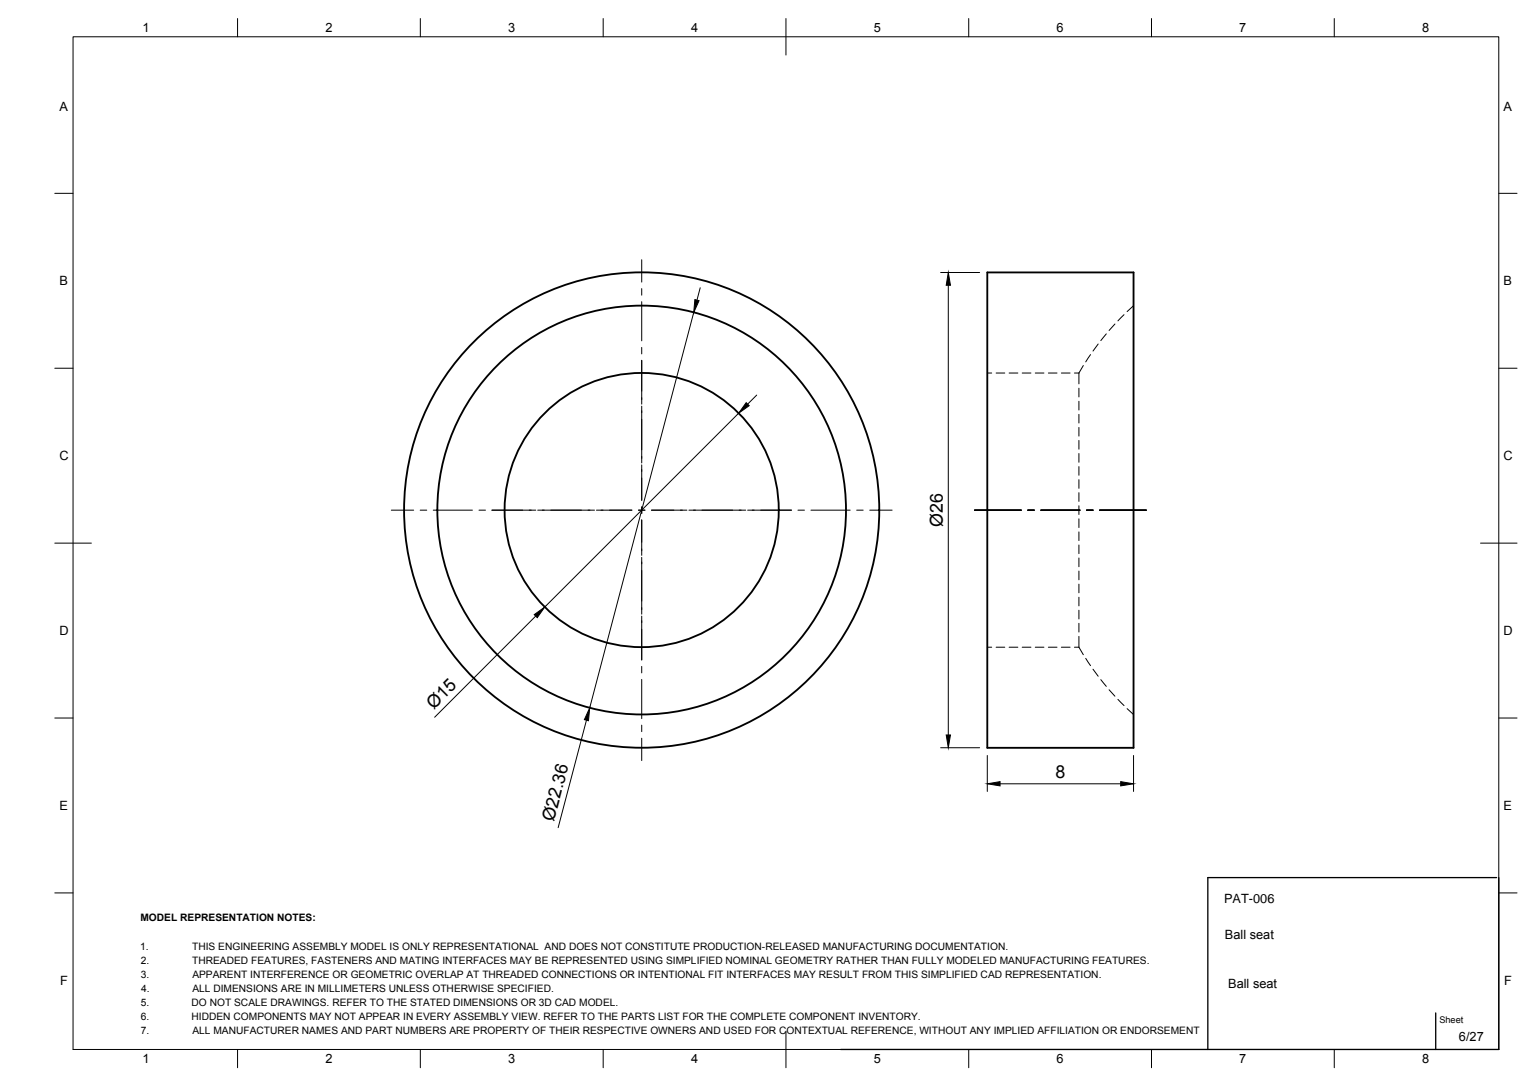
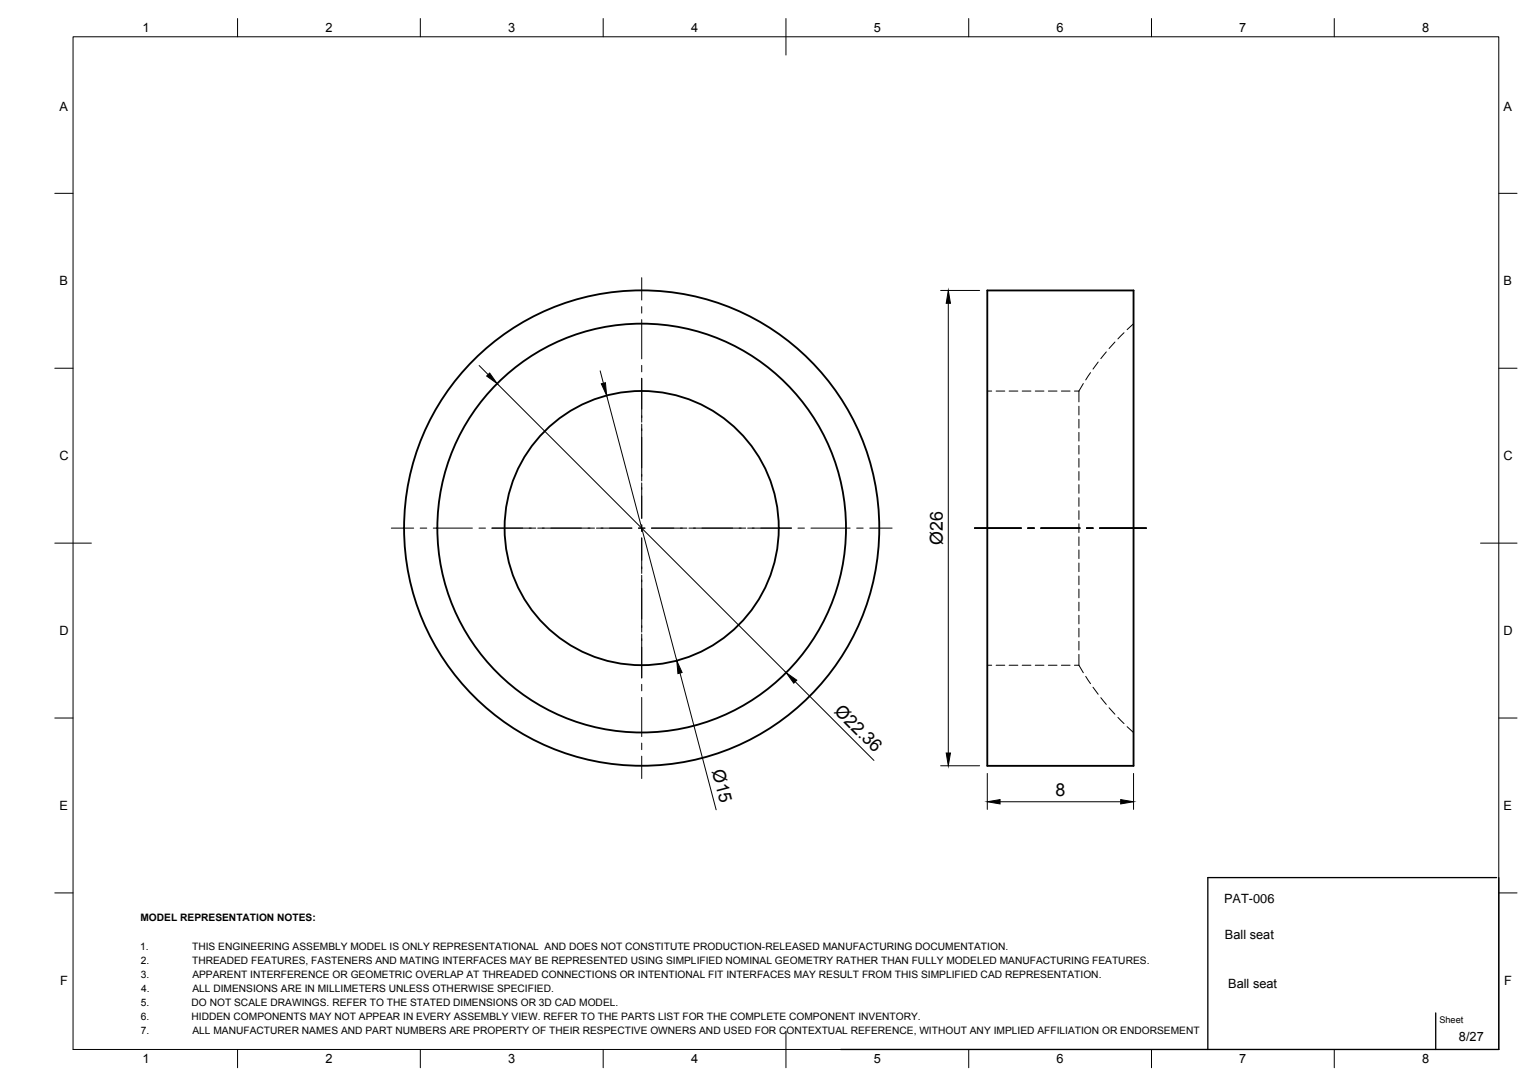
ISO-10303-21;
HEADER;
/* Generated by software containing ST-Developer
 * from STEP Tools, Inc. (www.steptools.com) 
 */

FILE_DESCRIPTION(
/* description */ ('Ball-type isolation valve (generic)'),
/* implementation_level */ '2;1');

FILE_NAME(
/* name */ 'Ball seat.step',
/* time_stamp */ '2026-10-27T10:53:05-07:00',
/* author */ (''),
/* organization */ (''),
/* preprocessor_version */ 'ST-DEVELOPER v20.2',
/* originating_system */ 'Autodesk Translation Framework v15.17.0.0',
/* authorisation */ '');

FILE_SCHEMA (('AUTOMOTIVE_DESIGN { 1 0 10303 214 3 1 1 }'));
ENDSEC;

DATA;
#10=MECHANICAL_DESIGN_GEOMETRIC_PRESENTATION_REPRESENTATION('',(#278),#7425);
#226=SHAPE_REPRESENTATION_RELATIONSHIP('SRR','None',#7536,#252);
#252=ADVANCED_BREP_SHAPE_REPRESENTATION('',(#304),#7399);
#278=STYLED_ITEM('',(#7730),#304);
#304=MANIFOLD_SOLID_BREP('Body1',#4083);
#327=SPHERICAL_SURFACE('',#4444,1.5);
#345=FACE_BOUND('',#864,.T.);
#346=FACE_BOUND('',#868,.T.);
#347=FACE_BOUND('',#870,.T.);
#430=PLANE('',#4452);
#431=PLANE('',#4453);
#600=FACE_OUTER_BOUND('',#863,.T.);
#601=FACE_OUTER_BOUND('',#865,.T.);
#602=FACE_OUTER_BOUND('',#866,.T.);
#603=FACE_OUTER_BOUND('',#867,.T.);
#604=FACE_OUTER_BOUND('',#869,.T.);
#863=EDGE_LOOP('',(#2867));
#864=EDGE_LOOP('',(#2868));
#865=EDGE_LOOP('',(#2869,#2870,#2871,#2872));
#866=EDGE_LOOP('',(#2873,#2874,#2875,#2876));
#867=EDGE_LOOP('',(#2877));
#868=EDGE_LOOP('',(#2878));
#869=EDGE_LOOP('',(#2879));
#870=EDGE_LOOP('',(#2880));
#1190=LINE('',#6309,#1498);
#1191=LINE('',#6315,#1499);
#1498=VECTOR('',#5021,0.75);
#1499=VECTOR('',#5028,1.3);
#1802=CIRCLE('',#4445,1.11803398874989);
#1803=CIRCLE('',#4446,0.75);
#1804=CIRCLE('',#4448,0.75);
#1805=CIRCLE('',#4450,1.3);
#1806=CIRCLE('',#4451,1.3);
#1987=VERTEX_POINT('',#6303);
#1988=VERTEX_POINT('',#6305);
#1989=VERTEX_POINT('',#6308);
#1990=VERTEX_POINT('',#6312);
#1991=VERTEX_POINT('',#6314);
#2326=EDGE_CURVE('',#1987,#1987,#1802,.T.);
#2327=EDGE_CURVE('',#1988,#1988,#1803,.T.);
#2328=EDGE_CURVE('',#1988,#1989,#1190,.T.);
#2329=EDGE_CURVE('',#1989,#1989,#1804,.T.);
#2330=EDGE_CURVE('',#1990,#1990,#1805,.T.);
#2331=EDGE_CURVE('',#1990,#1991,#1191,.T.);
#2332=EDGE_CURVE('',#1991,#1991,#1806,.T.);
#2867=ORIENTED_EDGE('',*,*,#2326,.F.);
#2868=ORIENTED_EDGE('',*,*,#2327,.F.);
#2869=ORIENTED_EDGE('',*,*,#2327,.T.);
#2870=ORIENTED_EDGE('',*,*,#2328,.T.);
#2871=ORIENTED_EDGE('',*,*,#2329,.T.);
#2872=ORIENTED_EDGE('',*,*,#2328,.F.);
#2873=ORIENTED_EDGE('',*,*,#2330,.F.);
#2874=ORIENTED_EDGE('',*,*,#2331,.T.);
#2875=ORIENTED_EDGE('',*,*,#2332,.T.);
#2876=ORIENTED_EDGE('',*,*,#2331,.F.);
#2877=ORIENTED_EDGE('',*,*,#2330,.T.);
#2878=ORIENTED_EDGE('',*,*,#2326,.T.);
#2879=ORIENTED_EDGE('',*,*,#2332,.F.);
#2880=ORIENTED_EDGE('',*,*,#2329,.F.);
#3774=CYLINDRICAL_SURFACE('',#4447,0.75);
#3775=CYLINDRICAL_SURFACE('',#4449,1.3);
#3854=ADVANCED_FACE('',(#600,#345),#327,.F.);
#3855=ADVANCED_FACE('',(#601),#3774,.F.);
#3856=ADVANCED_FACE('',(#602),#3775,.T.);
#3857=ADVANCED_FACE('',(#603,#346),#430,.T.);
#3858=ADVANCED_FACE('',(#604,#347),#431,.F.);
#4083=CLOSED_SHELL('',(#3854,#3855,#3856,#3857,#3858));
#4443=AXIS2_PLACEMENT_3D('',#6301,#5011,#5012);
#4444=AXIS2_PLACEMENT_3D('',#6302,#5013,#5014);
#4445=AXIS2_PLACEMENT_3D('',#6304,#5015,#5016);
#4446=AXIS2_PLACEMENT_3D('',#6306,#5017,#5018);
#4447=AXIS2_PLACEMENT_3D('',#6307,#5019,#5020);
#4448=AXIS2_PLACEMENT_3D('',#6310,#5022,#5023);
#4449=AXIS2_PLACEMENT_3D('',#6311,#5024,#5025);
#4450=AXIS2_PLACEMENT_3D('',#6313,#5026,#5027);
#4451=AXIS2_PLACEMENT_3D('',#6316,#5029,#5030);
#4452=AXIS2_PLACEMENT_3D('',#6317,#5031,#5032);
#4453=AXIS2_PLACEMENT_3D('',#6318,#5033,#5034);
#5011=DIRECTION('axis',(0.,0.,1.));
#5012=DIRECTION('refdir',(1.,0.,0.));
#5013=DIRECTION('center_axis',(6.12323399573677E-17,0.,1.));
#5014=DIRECTION('ref_axis',(1.,0.,0.));
#5015=DIRECTION('center_axis',(0.,-1.,0.));
#5016=DIRECTION('ref_axis',(0.,0.,-1.));
#5017=DIRECTION('center_axis',(0.,1.,0.));
#5018=DIRECTION('ref_axis',(1.,0.,0.));
#5019=DIRECTION('center_axis',(0.,1.,0.));
#5020=DIRECTION('ref_axis',(1.,0.,0.));
#5021=DIRECTION('',(0.,-1.,0.));
#5022=DIRECTION('center_axis',(0.,-1.,0.));
#5023=DIRECTION('ref_axis',(1.,0.,0.));
#5024=DIRECTION('center_axis',(0.,1.,0.));
#5025=DIRECTION('ref_axis',(1.,0.,0.));
#5026=DIRECTION('center_axis',(0.,1.,0.));
#5027=DIRECTION('ref_axis',(1.,0.,0.));
#5028=DIRECTION('',(0.,-1.,0.));
#5029=DIRECTION('center_axis',(0.,1.,0.));
#5030=DIRECTION('ref_axis',(1.,0.,0.));
#5031=DIRECTION('center_axis',(0.,1.,0.));
#5032=DIRECTION('ref_axis',(1.,0.,0.));
#5033=DIRECTION('center_axis',(0.,1.,0.));
#5034=DIRECTION('ref_axis',(1.,0.,0.));
#6301=CARTESIAN_POINT('',(0.,0.,0.));
#6302=CARTESIAN_POINT('Origin',(0.,0.,5.));
#6303=CARTESIAN_POINT('',(-1.36919674566051E-16,-1.,6.11803398874989));
#6304=CARTESIAN_POINT('Origin',(0.,-1.,5.));
#6305=CARTESIAN_POINT('',(-0.75,-1.29903810567666,5.));
#6306=CARTESIAN_POINT('Origin',(0.,-1.29903810567666,5.));
#6307=CARTESIAN_POINT('Origin',(0.,-1.8,5.));
#6308=CARTESIAN_POINT('',(-0.75,-1.8,5.));
#6309=CARTESIAN_POINT('',(-0.75,-1.8,5.));
#6310=CARTESIAN_POINT('Origin',(0.,-1.8,5.));
#6311=CARTESIAN_POINT('Origin',(0.,-1.8,5.));
#6312=CARTESIAN_POINT('',(-1.3,-1.,5.));
#6313=CARTESIAN_POINT('Origin',(0.,-1.,5.));
#6314=CARTESIAN_POINT('',(-1.3,-1.8,5.));
#6315=CARTESIAN_POINT('',(-1.3,-1.8,5.));
#6316=CARTESIAN_POINT('Origin',(0.,-1.8,5.));
#6317=CARTESIAN_POINT('Origin',(0.,-1.,5.));
#6318=CARTESIAN_POINT('Origin',(0.,-1.8,5.));
#7369=UNCERTAINTY_MEASURE_WITH_UNIT(LENGTH_MEASURE(0.001),#7426,
'DISTANCE_ACCURACY_VALUE',
'Maximum model space distance between geometric entities at asserted c
onnectivities');
#7395=UNCERTAINTY_MEASURE_WITH_UNIT(LENGTH_MEASURE(0.001),#7426,
'DISTANCE_ACCURACY_VALUE',
'Maximum model space distance between geometric entities at asserted c
onnectivities');
#7399=(
GEOMETRIC_REPRESENTATION_CONTEXT(3)
GLOBAL_UNCERTAINTY_ASSIGNED_CONTEXT((#7369))
GLOBAL_UNIT_ASSIGNED_CONTEXT((#7426,#7428,#7429))
REPRESENTATION_CONTEXT('','3D')
);
#7425=(
GEOMETRIC_REPRESENTATION_CONTEXT(3)
GLOBAL_UNCERTAINTY_ASSIGNED_CONTEXT((#7395))
GLOBAL_UNIT_ASSIGNED_CONTEXT((#7426,#7428,#7429))
REPRESENTATION_CONTEXT('','3D')
);
#7426=(
LENGTH_UNIT()
NAMED_UNIT(*)
SI_UNIT(.CENTI.,.METRE.)
);
#7428=(
NAMED_UNIT(*)
PLANE_ANGLE_UNIT()
SI_UNIT($,.RADIAN.)
);
#7429=(
NAMED_UNIT(*)
SI_UNIT($,.STERADIAN.)
SOLID_ANGLE_UNIT()
);
#7433=SHAPE_DEFINITION_REPRESENTATION(#7462,#7536);
#7462=PRODUCT_DEFINITION_SHAPE('',$,#7566);
#7536=SHAPE_REPRESENTATION('',(#4443),#7399);
#7562=PRODUCT_DEFINITION_CONTEXT('part definition',#7651,'design');
#7566=PRODUCT_DEFINITION('Ball seat','Ball seat',#7595,#7562);
#7595=PRODUCT_DEFINITION_FORMATION('',$,#7656);
#7651=APPLICATION_CONTEXT(
'Core Data for Automotive Mechanical Design Process');
#7652=PRODUCT_CONTEXT('part definition',#7651,'mechanical');
#7656=PRODUCT('Ball seat','Ball seat','Ball seat',(#7652));
#7724=COLOUR_RGB('Light Blue',0.38,0.62,0.78);
#7725=FILL_AREA_STYLE_COLOUR('',#7724);
#7726=FILL_AREA_STYLE('',(#7725));
#7727=SURFACE_STYLE_FILL_AREA(#7726);
#7728=SURFACE_SIDE_STYLE('',(#7727));
#7729=SURFACE_STYLE_USAGE(.BOTH.,#7728);
#7730=PRESENTATION_STYLE_ASSIGNMENT((#7729));
ENDSEC;
END-ISO-10303-21;
